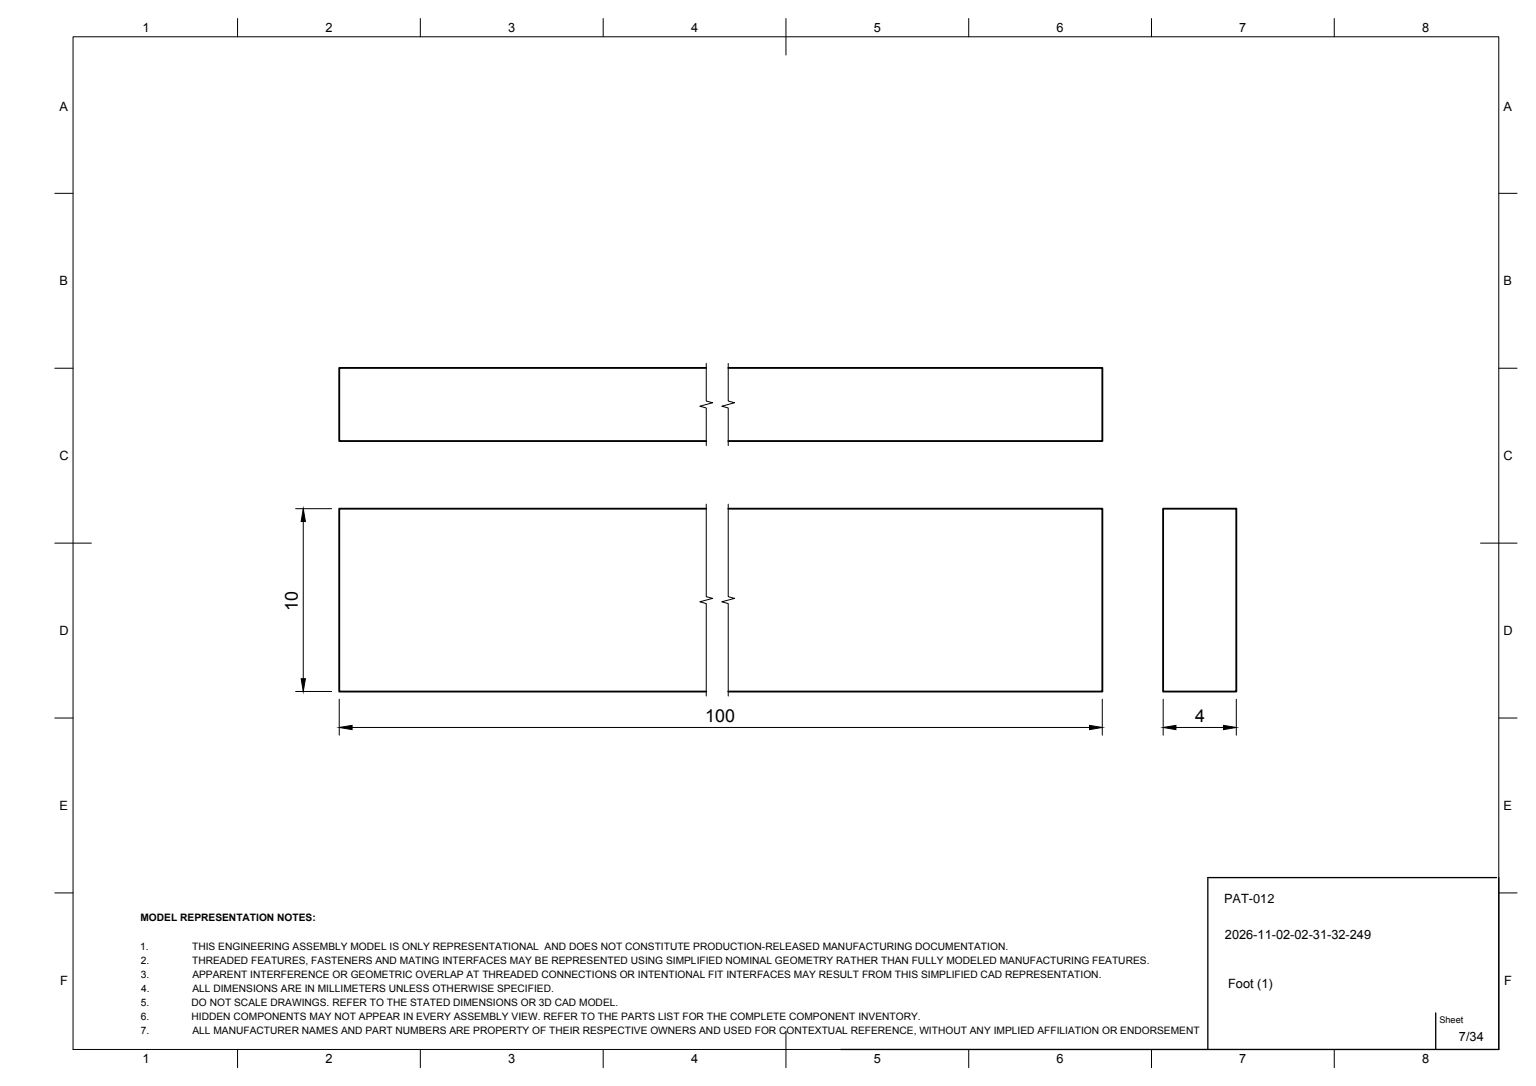
ISO-10303-21;
HEADER;
/* Generated by software containing ST-Developer
 * from STEP Tools, Inc. (www.steptools.com) 
 */

FILE_DESCRIPTION(
/* description */ ('Belt tensioner idler arm'),
/* implementation_level */ '2;1');

FILE_NAME(
/* name */ 'Foot (1).step',
/* time_stamp */ '2026-10-28T03:22:15-07:00',
/* author */ (''),
/* organization */ (''),
/* preprocessor_version */ 'ST-DEVELOPER v20.2',
/* originating_system */ 'Autodesk Translation Framework v15.17.0.0',
/* authorisation */ '');

FILE_SCHEMA (('AUTOMOTIVE_DESIGN { 1 0 10303 214 3 1 1 }'));
ENDSEC;

DATA;
#10=MECHANICAL_DESIGN_GEOMETRIC_PRESENTATION_REPRESENTATION('',(#449),#12779);
#381=SHAPE_REPRESENTATION_RELATIONSHIP('SRR','None',#12927,#415);
#415=ADVANCED_BREP_SHAPE_REPRESENTATION('',(#491),#12744);
#449=STYLED_ITEM('',(#13198),#491);
#491=MANIFOLD_SOLID_BREP('Body1',#6183);
#675=PLANE('',#6634);
#676=PLANE('',#6635);
#677=PLANE('',#6636);
#678=PLANE('',#6637);
#679=PLANE('',#6638);
#680=PLANE('',#6639);
#854=FACE_OUTER_BOUND('',#1231,.T.);
#855=FACE_OUTER_BOUND('',#1232,.T.);
#856=FACE_OUTER_BOUND('',#1233,.T.);
#857=FACE_OUTER_BOUND('',#1234,.T.);
#858=FACE_OUTER_BOUND('',#1235,.T.);
#859=FACE_OUTER_BOUND('',#1236,.T.);
#1231=EDGE_LOOP('',(#4164,#4165,#4166,#4167));
#1232=EDGE_LOOP('',(#4168,#4169,#4170,#4171));
#1233=EDGE_LOOP('',(#4172,#4173,#4174,#4175));
#1234=EDGE_LOOP('',(#4176,#4177,#4178,#4179));
#1235=EDGE_LOOP('',(#4180,#4181,#4182,#4183));
#1236=EDGE_LOOP('',(#4184,#4185,#4186,#4187));
#1736=LINE('',#9534,#2085);
#1737=LINE('',#9536,#2086);
#1738=LINE('',#9538,#2087);
#1739=LINE('',#9539,#2088);
#1740=LINE('',#9542,#2089);
#1741=LINE('',#9544,#2090);
#1742=LINE('',#9545,#2091);
#1743=LINE('',#9548,#2092);
#1744=LINE('',#9550,#2093);
#1745=LINE('',#9551,#2094);
#1746=LINE('',#9553,#2095);
#1747=LINE('',#9554,#2096);
#2085=VECTOR('',#7528,1.);
#2086=VECTOR('',#7529,1.);
#2087=VECTOR('',#7530,1.);
#2088=VECTOR('',#7531,1.);
#2089=VECTOR('',#7534,1.);
#2090=VECTOR('',#7535,1.);
#2091=VECTOR('',#7536,1.);
#2092=VECTOR('',#7539,1.);
#2093=VECTOR('',#7540,1.);
#2094=VECTOR('',#7541,1.);
#2095=VECTOR('',#7544,1.);
#2096=VECTOR('',#7545,1.);
#2795=VERTEX_POINT('',#9532);
#2796=VERTEX_POINT('',#9533);
#2797=VERTEX_POINT('',#9535);
#2798=VERTEX_POINT('',#9537);
#2799=VERTEX_POINT('',#9541);
#2800=VERTEX_POINT('',#9543);
#2801=VERTEX_POINT('',#9547);
#2802=VERTEX_POINT('',#9549);
#3337=EDGE_CURVE('',#2795,#2796,#1736,.T.);
#3338=EDGE_CURVE('',#2796,#2797,#1737,.T.);
#3339=EDGE_CURVE('',#2798,#2797,#1738,.T.);
#3340=EDGE_CURVE('',#2795,#2798,#1739,.T.);
#3341=EDGE_CURVE('',#2799,#2795,#1740,.T.);
#3342=EDGE_CURVE('',#2800,#2798,#1741,.T.);
#3343=EDGE_CURVE('',#2799,#2800,#1742,.T.);
#3344=EDGE_CURVE('',#2801,#2799,#1743,.T.);
#3345=EDGE_CURVE('',#2802,#2800,#1744,.T.);
#3346=EDGE_CURVE('',#2801,#2802,#1745,.T.);
#3347=EDGE_CURVE('',#2796,#2801,#1746,.T.);
#3348=EDGE_CURVE('',#2797,#2802,#1747,.T.);
#4164=ORIENTED_EDGE('',*,*,#3337,.T.);
#4165=ORIENTED_EDGE('',*,*,#3338,.T.);
#4166=ORIENTED_EDGE('',*,*,#3339,.F.);
#4167=ORIENTED_EDGE('',*,*,#3340,.F.);
#4168=ORIENTED_EDGE('',*,*,#3341,.T.);
#4169=ORIENTED_EDGE('',*,*,#3340,.T.);
#4170=ORIENTED_EDGE('',*,*,#3342,.F.);
#4171=ORIENTED_EDGE('',*,*,#3343,.F.);
#4172=ORIENTED_EDGE('',*,*,#3344,.T.);
#4173=ORIENTED_EDGE('',*,*,#3343,.T.);
#4174=ORIENTED_EDGE('',*,*,#3345,.F.);
#4175=ORIENTED_EDGE('',*,*,#3346,.F.);
#4176=ORIENTED_EDGE('',*,*,#3347,.T.);
#4177=ORIENTED_EDGE('',*,*,#3346,.T.);
#4178=ORIENTED_EDGE('',*,*,#3348,.F.);
#4179=ORIENTED_EDGE('',*,*,#3338,.F.);
#4180=ORIENTED_EDGE('',*,*,#3348,.T.);
#4181=ORIENTED_EDGE('',*,*,#3345,.T.);
#4182=ORIENTED_EDGE('',*,*,#3342,.T.);
#4183=ORIENTED_EDGE('',*,*,#3339,.T.);
#4184=ORIENTED_EDGE('',*,*,#3347,.F.);
#4185=ORIENTED_EDGE('',*,*,#3337,.F.);
#4186=ORIENTED_EDGE('',*,*,#3341,.F.);
#4187=ORIENTED_EDGE('',*,*,#3344,.F.);
#5831=ADVANCED_FACE('',(#854),#675,.T.);
#5832=ADVANCED_FACE('',(#855),#676,.T.);
#5833=ADVANCED_FACE('',(#856),#677,.T.);
#5834=ADVANCED_FACE('',(#857),#678,.T.);
#5835=ADVANCED_FACE('',(#858),#679,.T.);
#5836=ADVANCED_FACE('',(#859),#680,.F.);
#6183=CLOSED_SHELL('',(#5831,#5832,#5833,#5834,#5835,#5836));
#6633=AXIS2_PLACEMENT_3D('',#9530,#7524,#7525);
#6634=AXIS2_PLACEMENT_3D('',#9531,#7526,#7527);
#6635=AXIS2_PLACEMENT_3D('',#9540,#7532,#7533);
#6636=AXIS2_PLACEMENT_3D('',#9546,#7537,#7538);
#6637=AXIS2_PLACEMENT_3D('',#9552,#7542,#7543);
#6638=AXIS2_PLACEMENT_3D('',#9555,#7546,#7547);
#6639=AXIS2_PLACEMENT_3D('',#9556,#7548,#7549);
#7524=DIRECTION('axis',(0.,0.,1.));
#7525=DIRECTION('refdir',(1.,0.,0.));
#7526=DIRECTION('center_axis',(0.,1.,0.));
#7527=DIRECTION('ref_axis',(-1.,0.,0.));
#7528=DIRECTION('',(-1.,0.,0.));
#7529=DIRECTION('',(0.,0.,1.));
#7530=DIRECTION('',(-1.,0.,0.));
#7531=DIRECTION('',(0.,0.,1.));
#7532=DIRECTION('center_axis',(1.,0.,0.));
#7533=DIRECTION('ref_axis',(0.,1.,0.));
#7534=DIRECTION('',(0.,1.,0.));
#7535=DIRECTION('',(0.,1.,0.));
#7536=DIRECTION('',(0.,0.,1.));
#7537=DIRECTION('center_axis',(0.,-1.,0.));
#7538=DIRECTION('ref_axis',(1.,0.,0.));
#7539=DIRECTION('',(1.,0.,0.));
#7540=DIRECTION('',(1.,0.,0.));
#7541=DIRECTION('',(0.,0.,1.));
#7542=DIRECTION('center_axis',(-1.,0.,0.));
#7543=DIRECTION('ref_axis',(0.,-1.,0.));
#7544=DIRECTION('',(0.,-1.,0.));
#7545=DIRECTION('',(0.,-1.,0.));
#7546=DIRECTION('center_axis',(0.,0.,1.));
#7547=DIRECTION('ref_axis',(1.,0.,0.));
#7548=DIRECTION('center_axis',(0.,0.,1.));
#7549=DIRECTION('ref_axis',(1.,0.,0.));
#9530=CARTESIAN_POINT('',(0.,0.,0.));
#9531=CARTESIAN_POINT('Origin',(12.,5.5,-1.4));
#9532=CARTESIAN_POINT('',(12.,5.5,-1.4));
#9533=CARTESIAN_POINT('',(11.,5.5,-1.4));
#9534=CARTESIAN_POINT('',(12.,5.5,-1.4));
#9535=CARTESIAN_POINT('',(11.,5.5,-1.));
#9536=CARTESIAN_POINT('',(11.,5.5,-1.4));
#9537=CARTESIAN_POINT('',(12.,5.5,-1.));
#9538=CARTESIAN_POINT('',(12.,5.5,-1.));
#9539=CARTESIAN_POINT('',(12.,5.5,-1.4));
#9540=CARTESIAN_POINT('Origin',(12.,-4.5,-1.4));
#9541=CARTESIAN_POINT('',(12.,-4.5,-1.4));
#9542=CARTESIAN_POINT('',(12.,-4.5,-1.4));
#9543=CARTESIAN_POINT('',(12.,-4.5,-1.));
#9544=CARTESIAN_POINT('',(12.,-4.5,-1.));
#9545=CARTESIAN_POINT('',(12.,-4.5,-1.4));
#9546=CARTESIAN_POINT('Origin',(11.,-4.5,-1.4));
#9547=CARTESIAN_POINT('',(11.,-4.5,-1.4));
#9548=CARTESIAN_POINT('',(11.,-4.5,-1.4));
#9549=CARTESIAN_POINT('',(11.,-4.5,-1.));
#9550=CARTESIAN_POINT('',(11.,-4.5,-1.));
#9551=CARTESIAN_POINT('',(11.,-4.5,-1.4));
#9552=CARTESIAN_POINT('Origin',(11.,5.5,-1.4));
#9553=CARTESIAN_POINT('',(11.,5.5,-1.4));
#9554=CARTESIAN_POINT('',(11.,5.5,-1.));
#9555=CARTESIAN_POINT('Origin',(11.5,0.5,-1.));
#9556=CARTESIAN_POINT('Origin',(11.5,0.5,-1.4));
#12704=UNCERTAINTY_MEASURE_WITH_UNIT(LENGTH_MEASURE(0.001),#12780,
'DISTANCE_ACCURACY_VALUE',
'Maximum model space distance between geometric entities at asserted c
onnectivities');
#12739=UNCERTAINTY_MEASURE_WITH_UNIT(LENGTH_MEASURE(0.001),#12780,
'DISTANCE_ACCURACY_VALUE',
'Maximum model space distance between geometric entities at asserted c
onnectivities');
#12744=(
GEOMETRIC_REPRESENTATION_CONTEXT(3)
GLOBAL_UNCERTAINTY_ASSIGNED_CONTEXT((#12704))
GLOBAL_UNIT_ASSIGNED_CONTEXT((#12780,#12782,#12783))
REPRESENTATION_CONTEXT('','3D')
);
#12779=(
GEOMETRIC_REPRESENTATION_CONTEXT(3)
GLOBAL_UNCERTAINTY_ASSIGNED_CONTEXT((#12739))
GLOBAL_UNIT_ASSIGNED_CONTEXT((#12780,#12782,#12783))
REPRESENTATION_CONTEXT('','3D')
);
#12780=(
LENGTH_UNIT()
NAMED_UNIT(*)
SI_UNIT(.CENTI.,.METRE.)
);
#12782=(
NAMED_UNIT(*)
PLANE_ANGLE_UNIT()
SI_UNIT($,.RADIAN.)
);
#12783=(
NAMED_UNIT(*)
SI_UNIT($,.STERADIAN.)
SOLID_ANGLE_UNIT()
);
#12788=SHAPE_DEFINITION_REPRESENTATION(#12827,#12927);
#12827=PRODUCT_DEFINITION_SHAPE('',$,#12967);
#12927=SHAPE_REPRESENTATION('',(#6633),#12744);
#12962=PRODUCT_DEFINITION_CONTEXT('part definition',#13081,'design');
#12967=PRODUCT_DEFINITION('Foot (1)','Foot (1)',#13006,#12962);
#13006=PRODUCT_DEFINITION_FORMATION('',$,#13087);
#13081=APPLICATION_CONTEXT(
'Core Data for Automotive Mechanical Design Process');
#13082=PRODUCT_CONTEXT('part definition',#13081,'mechanical');
#13087=PRODUCT('Foot (1)','Foot (1)','Foot (1)',(#13082));
#13192=COLOUR_RGB('Off White',0.89,0.88,0.83);
#13193=FILL_AREA_STYLE_COLOUR('',#13192);
#13194=FILL_AREA_STYLE('',(#13193));
#13195=SURFACE_STYLE_FILL_AREA(#13194);
#13196=SURFACE_SIDE_STYLE('',(#13195));
#13197=SURFACE_STYLE_USAGE(.BOTH.,#13196);
#13198=PRESENTATION_STYLE_ASSIGNMENT((#13197));
ENDSEC;
END-ISO-10303-21;
